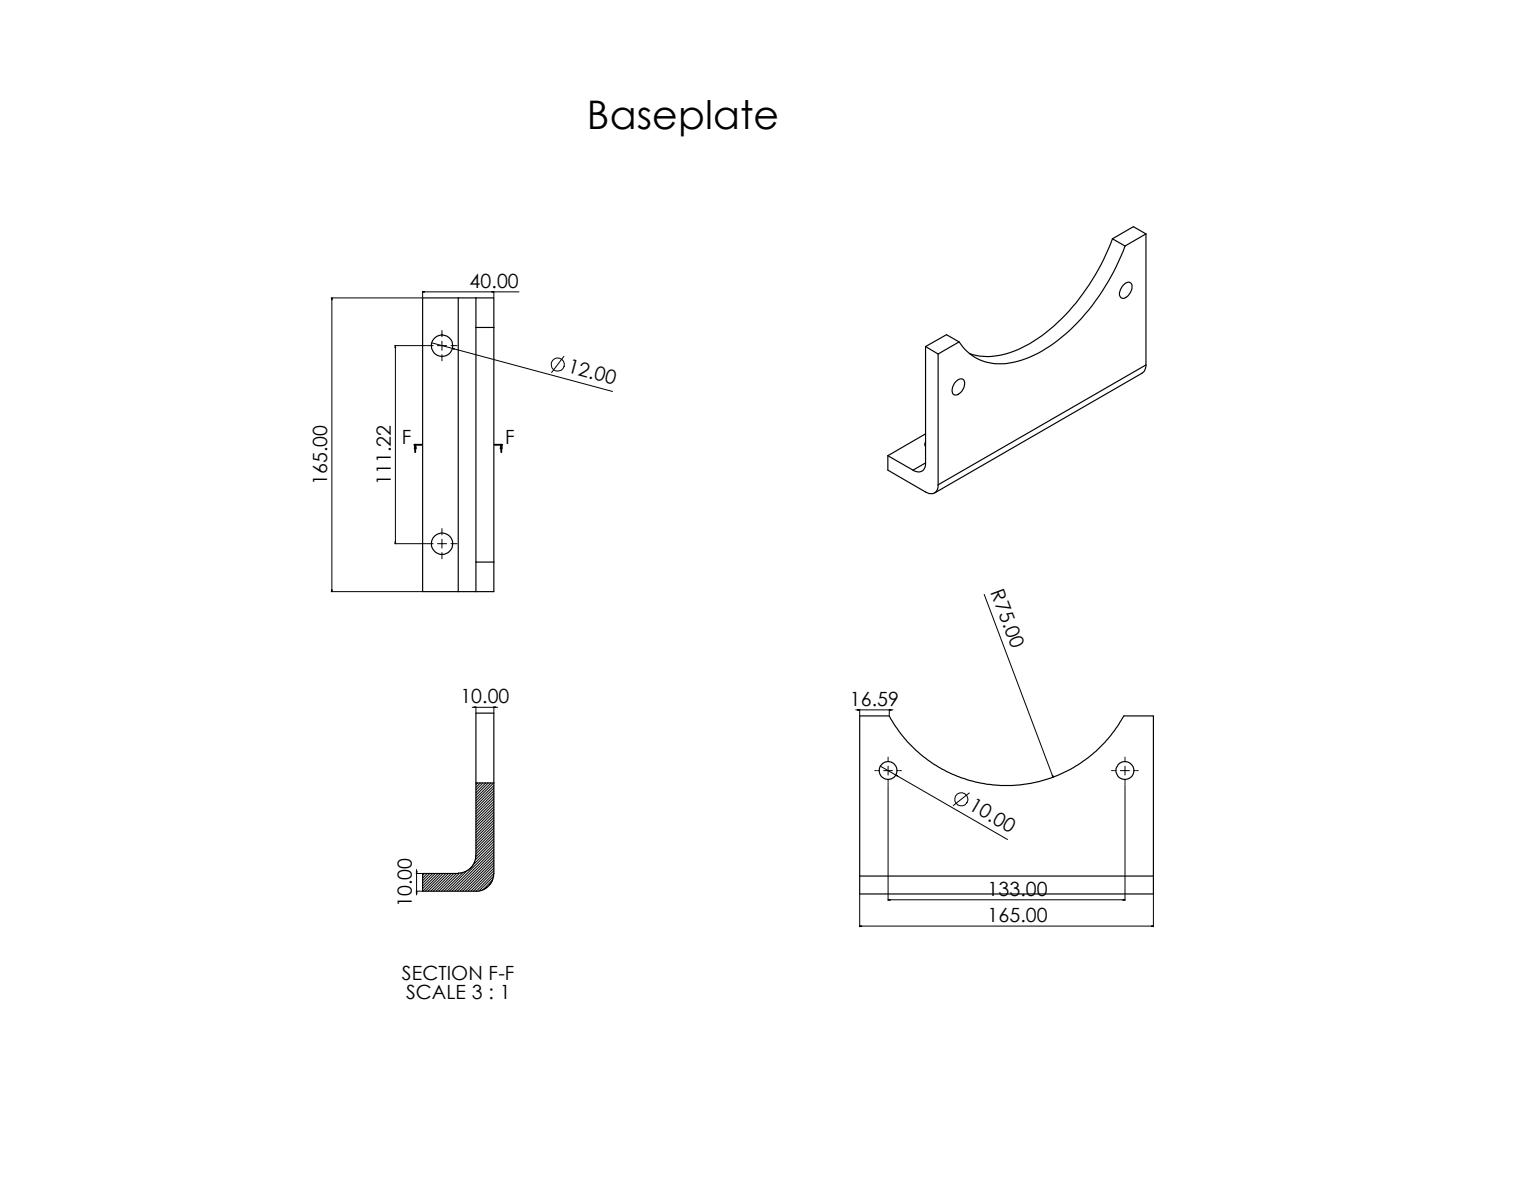
ISO-10303-21;
HEADER;
FILE_DESCRIPTION (('STEP AP214'),
    '1' );
FILE_NAME ('Baseplate.step',
    '2026-10-27T19:20:31',
    ( '' ),
    ( '' ),
    'SwSTEP 2.0',
    'SolidWorks 2025',
    '' );
FILE_SCHEMA (( 'AUTOMOTIVE_DESIGN' ));
ENDSEC;

DATA;
#22=DIRECTION ( 'NONE',  ( 0.000000000000000000, 0.000000000000000000, 1.000000000000000000 ) ) ;
#38=DIRECTION ( 'NONE',  ( -1.836970198721030427E-16, 1.000000000000000000, -1.682156097916904327E-16 ) ) ;
#169=DIRECTION ( 'NONE',  ( 0.000000000000000000, -1.000000000000000000, 0.000000000000000000 ) ) ;
#190=EDGE_CURVE ( 'NONE', #22454, #4199, #20086, .T. ) ;
#222=( GEOMETRIC_REPRESENTATION_CONTEXT ( 3 ) GLOBAL_UNCERTAINTY_ASSIGNED_CONTEXT ( ( #25788 ) ) GLOBAL_UNIT_ASSIGNED_CONTEXT ( ( #19170, #953, #19420 ) ) REPRESENTATION_CONTEXT ( 'NONE', 'WORKASPACE' ) );
#232=CIRCLE ( 'NONE', #10863, 5.000000000000004441 ) ;
#247=AXIS2_PLACEMENT_3D ( 'NONE', #22404, #17983, #169 ) ;
#303=CARTESIAN_POINT ( 'NONE',  ( 190.0000000000000000, 2.476104986517924766E-14, 4.683861624749757595E-30 ) ) ;
#341=CARTESIAN_POINT ( 'NONE',  ( 180.0000000000000000, -61.50000000000001421, 66.50000000000005684 ) ) ;
#389=EDGE_CURVE ( 'NONE', #22079, #14258, #2389, .T. ) ;
#393=VECTOR ( 'NONE', #2972, 1000.000000000000000 ) ;
#453=CARTESIAN_POINT ( 'NONE',  ( 150.0000000000000284, -135.7889608577475258, -82.49999999999998579 ) ) ;
#459=LINE ( 'NONE', #6827, #7636 ) ;
#575=PLANE ( 'NONE',  #7887 ) ;
#693=EDGE_LOOP ( 'NONE', ( #13184, #9222, #23705, #13464 ) ) ;
#761=ORIENTED_EDGE ( 'NONE', *, *, #11193, .T. ) ;
#786=ORIENTED_EDGE ( 'NONE', *, *, #16697, .F. ) ;
#795=EDGE_CURVE ( 'NONE', #24980, #854, #10474, .T. ) ;
#848=LINE ( 'NONE', #8957, #8452 ) ;
#854=VERTEX_POINT ( 'NONE', #22798 ) ;
#878=CARTESIAN_POINT ( 'NONE',  ( 160.9163046357249129, -135.7889608577475542, -55.61140153332245006 ) ) ;
#890=ORIENTED_EDGE ( 'NONE', *, *, #2098, .F. ) ;
#953=( NAMED_UNIT ( * ) PLANE_ANGLE_UNIT ( ) SI_UNIT ( $, .RADIAN. ) );
#983=DIRECTION ( 'NONE',  ( 1.000000000000000000, 1.836970198721030427E-16, -0.000000000000000000 ) ) ;
#1049=ORIENTED_EDGE ( 'NONE', *, *, #22501, .T. ) ;
#1059=LINE ( 'NONE', #1190, #21088 ) ;
#1076=DIRECTION ( 'NONE',  ( -1.303213150798907793E-16, 1.000000000000000000, -1.682156097916904081E-16 ) ) ;
#1086=VECTOR ( 'NONE', #8418, 1000.000000000000000 ) ;
#1119=ORIENTED_EDGE ( 'NONE', *, *, #1862, .F. ) ;
#1146=LINE ( 'NONE', #13362, #1967 ) ;
#1164=CARTESIAN_POINT ( 'NONE',  ( 160.9163046357249129, -135.7889608577475542, -61.61140153332246427 ) ) ;
#1190=CARTESIAN_POINT ( 'NONE',  ( 160.9163046357249129, -205.7889608577475542, 61.61140153332252112 ) ) ;
#1237=ORIENTED_EDGE ( 'NONE', *, *, #12981, .F. ) ;
#1245=EDGE_LOOP ( 'NONE', ( #24383, #1697, #17206, #26322 ) ) ;
#1290=DIRECTION ( 'NONE',  ( -1.000000000000000000, -1.836970198721030427E-16, 0.000000000000000000 ) ) ;
#1371=CYLINDRICAL_SURFACE ( 'NONE', #14023, 5.000000000000004441 ) ;
#1437=AXIS2_PLACEMENT_3D ( 'NONE', #19135, #5044, #3043 ) ;
#1446=LINE ( 'NONE', #23782, #16395 ) ;
#1451=FACE_OUTER_BOUND ( 'NONE', #20749, .T. ) ;
#1462=DIRECTION ( 'NONE',  ( 1.000000000000000000, 1.836970198721030427E-16, -0.000000000000000000 ) ) ;
#1499=EDGE_CURVE ( 'NONE', #1963, #23636, #7438, .T. ) ;
#1524=CIRCLE ( 'NONE', #247, 9.999999999999994671 ) ;
#1616=DIRECTION ( 'NONE',  ( -5.098616525425841937E-32, 2.775557561562890858E-16, 1.000000000000000000 ) ) ;
#1627=FACE_OUTER_BOUND ( 'NONE', #2486, .T. ) ;
#1641=AXIS2_PLACEMENT_3D ( 'NONE', #21190, #23317, #16661 ) ;
#1644=CARTESIAN_POINT ( 'NONE',  ( 180.0000000000000284, -125.7889608577475116, 82.50000000000001421 ) ) ;
#1661=ORIENTED_EDGE ( 'NONE', *, *, #9798, .F. ) ;
#1697=ORIENTED_EDGE ( 'NONE', *, *, #15786, .F. ) ;
#1720=SHAPE_DEFINITION_REPRESENTATION ( #22072, #14572 ) ;
#1730=CARTESIAN_POINT ( 'NONE',  ( 150.0000000000000284, -125.7889608577475116, 82.50000000000001421 ) ) ;
#1737=CIRCLE ( 'NONE', #16606, 6.000000000000005329 ) ;
#1764=ADVANCED_FACE ( 'NONE', ( #15599, #23724, #21735 ), #7614, .F. ) ;
#1799=CIRCLE ( 'NONE', #3481, 6.000000000000019540 ) ;
#1819=ADVANCED_FACE ( 'NONE', ( #21360 ), #3129, .F. ) ;
#1862=EDGE_CURVE ( 'NONE', #16337, #25804, #232, .T. ) ;
#1901=ORIENTED_EDGE ( 'NONE', *, *, #389, .F. ) ;
#1963=VERTEX_POINT ( 'NONE', #1164 ) ;
#1967=VECTOR ( 'NONE', #9633, 1000.000000000000000 ) ;
#1981=VECTOR ( 'NONE', #5648, 1000.000000000000000 ) ;
#1984=VERTEX_POINT ( 'NONE', #7261 ) ;
#1994=DIRECTION ( 'NONE',  ( 2.985653255390529422E-32, -4.182618615277681568E-16, 1.000000000000000000 ) ) ;
#2001=EDGE_CURVE ( 'NONE', #23636, #1963, #4068, .T. ) ;
#2032=CARTESIAN_POINT ( 'NONE',  ( 160.9163046357249129, -125.7889608577475684, -55.61140153332245006 ) ) ;
#2071=CARTESIAN_POINT ( 'NONE',  ( 180.0000000000000284, -115.7889608577475258, 82.50000000000000000 ) ) ;
#2098=EDGE_CURVE ( 'NONE', #3856, #1984, #3667, .T. ) ;
#2174=DIRECTION ( 'NONE',  ( 0.000000000000000000, 0.000000000000000000, 1.000000000000000000 ) ) ;
#2186=VECTOR ( 'NONE', #25982, 1000.000000000000000 ) ;
#2193=CIRCLE ( 'NONE', #17641, 10.00000000000000888 ) ;
#2273=PLANE ( 'NONE',  #23836 ) ;
#2302=DIRECTION ( 'NONE',  ( 1.000000000000000000, 1.836970198721030427E-16, -0.000000000000000000 ) ) ;
#2313=EDGE_CURVE ( 'NONE', #25993, #2419, #22542, .T. ) ;
#2389=CIRCLE ( 'NONE', #20666, 6.000000000000019540 ) ;
#2419=VERTEX_POINT ( 'NONE', #14277 ) ;
#2425=VERTEX_POINT ( 'NONE', #453 ) ;
#2486=EDGE_LOOP ( 'NONE', ( #15483, #4393, #761, #12919 ) ) ;
#2514=CARTESIAN_POINT ( 'NONE',  ( 190.0000000000000000, -66.50000000000001421, -66.50000000000005684 ) ) ;
#2541=DIRECTION ( 'NONE',  ( 0.000000000000000000, -1.000000000000000000, 0.000000000000000000 ) ) ;
#2542=CARTESIAN_POINT ( 'NONE',  ( 190.0000000000000284, -125.7889608577475400, 2.115966675574909200E-14 ) ) ;
#2598=ADVANCED_FACE ( 'NONE', ( #23153 ), #20895, .F. ) ;
#2627=AXIS2_PLACEMENT_3D ( 'NONE', #12406, #2302, #18529 ) ;
#2757=EDGE_LOOP ( 'NONE', ( #3114, #1049, #11674, #13097 ) ) ;
#2799=AXIS2_PLACEMENT_3D ( 'NONE', #21130, #9017, #25385 ) ;
#2813=PRODUCT_DEFINITION_FORMATION_WITH_SPECIFIED_SOURCE ( 'ANY', '', #15879, .NOT_KNOWN. ) ;
#2815=CARTESIAN_POINT ( 'NONE',  ( 180.0000000000000000, 2.292407966645821729E-14, 4.683861624749757595E-30 ) ) ;
#2925=CARTESIAN_POINT ( 'NONE',  ( 180.0000000000000284, -125.7889608577475684, -82.49999999999998579 ) ) ;
#2972=DIRECTION ( 'NONE',  ( -1.303213150798907793E-16, 1.000000000000000000, -1.682156097916904081E-16 ) ) ;
#2985=EDGE_CURVE ( 'NONE', #23734, #20976, #1059, .T. ) ;
#3043=DIRECTION ( 'NONE',  ( 0.000000000000000000, 0.000000000000000000, 1.000000000000000000 ) ) ;
#3114=ORIENTED_EDGE ( 'NONE', *, *, #15003, .T. ) ;
#3129=CYLINDRICAL_SURFACE ( 'NONE', #16804, 6.000000000000019540 ) ;
#3149=ADVANCED_FACE ( 'NONE', ( #9918 ), #11915, .F. ) ;
#3162=FACE_BOUND ( 'NONE', #7335, .T. ) ;
#3231=CARTESIAN_POINT ( 'NONE',  ( 180.0000000000000000, -66.50000000000001421, 66.50000000000005684 ) ) ;
#3239=VERTEX_POINT ( 'NONE', #4611 ) ;
#3268=AXIS2_PLACEMENT_3D ( 'NONE', #24504, #16507, #2541 ) ;
#3286=PLANE ( 'NONE',  #16622 ) ;
#3391=EDGE_CURVE ( 'NONE', #22320, #25804, #8962, .T. ) ;
#3481=AXIS2_PLACEMENT_3D ( 'NONE', #7276, #3549, #15638 ) ;
#3488=DIRECTION ( 'NONE',  ( 0.000000000000000000, 1.000000000000000000, 0.000000000000000000 ) ) ;
#3495=ORIENTED_EDGE ( 'NONE', *, *, #4923, .T. ) ;
#3511=CARTESIAN_POINT ( 'NONE',  ( 150.0000000000000284, -125.7889608577475116, 82.50000000000001421 ) ) ;
#3549=DIRECTION ( 'NONE',  ( -1.303213150798907793E-16, 1.000000000000000000, -1.682156097916904081E-16 ) ) ;
#3564=LINE ( 'NONE', #25933, #6385 ) ;
#3614=DIRECTION ( 'NONE',  ( -1.303213150798907793E-16, 1.000000000000000000, -1.682156097916904081E-16 ) ) ;
#3644=AXIS2_PLACEMENT_3D ( 'NONE', #26029, #19888, #19624 ) ;
#3654=AXIS2_PLACEMENT_3D ( 'NONE', #4347, #5933, #18024 ) ;
#3661=CARTESIAN_POINT ( 'NONE',  ( 180.0000000000000000, -35.78896085774750446, -65.91016826501511616 ) ) ;
#3667=LINE ( 'NONE', #5931, #9143 ) ;
#3723=VERTEX_POINT ( 'NONE', #7849 ) ;
#3849=CIRCLE ( 'NONE', #7183, 5.000000000000004441 ) ;
#3856=VERTEX_POINT ( 'NONE', #7413 ) ;
#3876=EDGE_CURVE ( 'NONE', #9443, #22454, #1446, .T. ) ;
#3925=CARTESIAN_POINT ( 'NONE',  ( 150.0000000000000284, -125.7889608577475116, 82.50000000000001421 ) ) ;
#3957=EDGE_LOOP ( 'NONE', ( #25081, #3495, #786, #25524, #5205, #9062, #4826, #21169 ) ) ;
#3989=ORIENTED_EDGE ( 'NONE', *, *, #9879, .F. ) ;
#4021=ORIENTED_EDGE ( 'NONE', *, *, #11906, .T. ) ;
#4064=( GEOMETRIC_REPRESENTATION_CONTEXT ( 3 ) GLOBAL_UNCERTAINTY_ASSIGNED_CONTEXT ( ( #15216 ) ) GLOBAL_UNIT_ASSIGNED_CONTEXT ( ( #10800, #10528, #18506 ) ) REPRESENTATION_CONTEXT ( 'NONE', 'WORKASPACE' ) );
#4068=CIRCLE ( 'NONE', #2799, 6.000000000000005329 ) ;
#4134=ORIENTED_EDGE ( 'NONE', *, *, #15447, .T. ) ;
#4137=DIRECTION ( 'NONE',  ( 0.000000000000000000, -1.682156097916903834E-16, -1.000000000000000000 ) ) ;
#4168=VERTEX_POINT ( 'NONE', #3925 ) ;
#4199=VERTEX_POINT ( 'NONE', #16543 ) ;
#4234=DIRECTION ( 'NONE',  ( -1.303213150798907793E-16, 1.000000000000000000, -1.682156097916904081E-16 ) ) ;
#4284=FACE_OUTER_BOUND ( 'NONE', #10394, .T. ) ;
#4347=CARTESIAN_POINT ( 'NONE',  ( 169.9999999999999716, -115.7889608577475258, 82.50000000000001421 ) ) ;
#4393=ORIENTED_EDGE ( 'NONE', *, *, #23125, .F. ) ;
#4439=CYLINDRICAL_SURFACE ( 'NONE', #5169, 74.99999999999995737 ) ;
#4459=EDGE_LOOP ( 'NONE', ( #13810, #22818, #22074, #18648 ) ) ;
#4495=DIRECTION ( 'NONE',  ( 1.000000000000000000, 1.303213150798907793E-16, 2.465190328815661892E-32 ) ) ;
#4549=LINE ( 'NONE', #14377, #15153 ) ;
#4571=CARTESIAN_POINT ( 'NONE',  ( 190.0000000000000000, 4.765939974807309500E-14, 82.49999999999997158 ) ) ;
#4580=DIRECTION ( 'NONE',  ( 1.000000000000000000, 1.303213150798907793E-16, 2.465190328815661892E-32 ) ) ;
#4604=ADVANCED_FACE ( 'NONE', ( #15815 ), #15950, .F. ) ;
#4611=CARTESIAN_POINT ( 'NONE',  ( 180.0000000000000284, -135.7889608577475542, -82.49999999999998579 ) ) ;
#4631=DIRECTION ( 'NONE',  ( 2.985653255390529422E-32, -4.182618615277681568E-16, 1.000000000000000000 ) ) ;
#4666=DIRECTION ( 'NONE',  ( 1.000000000000000000, 0.000000000000000000, -0.000000000000000000 ) ) ;
#4725=CARTESIAN_POINT ( 'NONE',  ( 160.9163046357249129, -125.7889608577475400, 55.61140153332248559 ) ) ;
#4826=ORIENTED_EDGE ( 'NONE', *, *, #15003, .F. ) ;
#4923=EDGE_CURVE ( 'NONE', #1984, #6082, #2193, .T. ) ;
#4973=EDGE_CURVE ( 'NONE', #9342, #8967, #1524, .T. ) ;
#5044=DIRECTION ( 'NONE',  ( -1.303213150798907793E-16, 1.000000000000000000, -1.682156097916904081E-16 ) ) ;
#5079=EDGE_LOOP ( 'NONE', ( #1119, #10639 ) ) ;
#5169=AXIS2_PLACEMENT_3D ( 'NONE', #10548, #21194, #9079 ) ;
#5180=AXIS2_PLACEMENT_3D ( 'NONE', #15679, #23804, #23309 ) ;
#5205=ORIENTED_EDGE ( 'NONE', *, *, #15010, .T. ) ;
#5263=ORIENTED_EDGE ( 'NONE', *, *, #25351, .T. ) ;
#5362=VERTEX_POINT ( 'NONE', #20369 ) ;
#5374=CARTESIAN_POINT ( 'NONE',  ( 160.9163046357249129, -125.7889608577475684, -61.61140153332246427 ) ) ;
#5379=DIRECTION ( 'NONE',  ( -1.000000000000000000, 0.000000000000000000, 0.000000000000000000 ) ) ;
#5505=DIRECTION ( 'NONE',  ( -1.836970198721030427E-16, 1.000000000000000000, -1.682156097916904327E-16 ) ) ;
#5624=DIRECTION ( 'NONE',  ( 1.000000000000000000, 1.303213150798907793E-16, 2.465190328815661892E-32 ) ) ;
#5648=DIRECTION ( 'NONE',  ( 1.303213150798907793E-16, -1.000000000000000000, 0.000000000000000000 ) ) ;
#5684=FACE_OUTER_BOUND ( 'NONE', #14455, .T. ) ;
#5699=PRODUCT_CONTEXT ( 'NONE', #16389, 'mechanical' ) ;
#5749=EDGE_CURVE ( 'NONE', #9443, #10429, #17877, .T. ) ;
#5767=DIRECTION ( 'NONE',  ( 0.000000000000000000, 0.000000000000000000, 1.000000000000000000 ) ) ;
#5770=VECTOR ( 'NONE', #24556, 1000.000000000000000 ) ;
#5864=DIRECTION ( 'NONE',  ( 0.000000000000000000, -4.182618615277681568E-16, 1.000000000000000000 ) ) ;
#5875=LINE ( 'NONE', #15974, #2186 ) ;
#5931=CARTESIAN_POINT ( 'NONE',  ( 180.0000000000000284, -135.7889608577475258, 82.50000000000001421 ) ) ;
#5933=DIRECTION ( 'NONE',  ( 4.657398277317546459E-32, -1.682156097916904081E-16, -1.000000000000000000 ) ) ;
#5949=CIRCLE ( 'NONE', #22097, 74.99999999999995737 ) ;
#5966=DIRECTION ( 'NONE',  ( -4.657398277317547006E-32, 1.682156097916904327E-16, 1.000000000000000000 ) ) ;
#5971=EDGE_CURVE ( 'NONE', #2425, #3856, #1146, .T. ) ;
#6082=VERTEX_POINT ( 'NONE', #13338 ) ;
#6100=DIRECTION ( 'NONE',  ( 0.000000000000000000, -4.182618615277681568E-16, -1.000000000000000000 ) ) ;
#6106=ORIENTED_EDGE ( 'NONE', *, *, #24953, .T. ) ;
#6111=CARTESIAN_POINT ( 'NONE',  ( 190.0000000000000000, -35.78896085774753288, -1.496915739050591872E-14 ) ) ;
#6142=DIRECTION ( 'NONE',  ( 0.000000000000000000, 0.000000000000000000, -1.000000000000000000 ) ) ;
#6240=EDGE_LOOP ( 'NONE', ( #1237, #23465, #23167, #18848 ) ) ;
#6283=CARTESIAN_POINT ( 'NONE',  ( 169.9999999999999716, -115.7889608577475542, -82.49999999999998579 ) ) ;
#6370=EDGE_CURVE ( 'NONE', #21146, #2419, #9439, .T. ) ;
#6385=VECTOR ( 'NONE', #24052, 1000.000000000000000 ) ;
#6386=DIRECTION ( 'NONE',  ( -1.836970198721030427E-16, 1.000000000000000000, 4.182618615277681568E-16 ) ) ;
#6460=VECTOR ( 'NONE', #12832, 1000.000000000000000 ) ;
#6476=CARTESIAN_POINT ( 'NONE',  ( 180.0000000000000000, -35.78896085774753288, -1.496915739050591872E-14 ) ) ;
#6530=ORIENTED_EDGE ( 'NONE', *, *, #15786, .T. ) ;
#6537=ORIENTED_EDGE ( 'NONE', *, *, #16385, .F. ) ;
#6548=DIRECTION ( 'NONE',  ( 0.000000000000000000, -1.000000000000000000, 0.000000000000000000 ) ) ;
#6553=CARTESIAN_POINT ( 'NONE',  ( 160.9163046357249129, -205.7889608577475542, -61.61140153332245006 ) ) ;
#6633=EDGE_CURVE ( 'NONE', #25845, #3723, #11178, .T. ) ;
#6677=DIRECTION ( 'NONE',  ( 1.303213150798907793E-16, -1.000000000000000000, 0.000000000000000000 ) ) ;
#6764=ORIENTED_EDGE ( 'NONE', *, *, #9798, .T. ) ;
#6805=DIRECTION ( 'NONE',  ( 7.916033913021854848E-32, -4.182618615277681568E-16, -1.000000000000000000 ) ) ;
#6827=CARTESIAN_POINT ( 'NONE',  ( 180.0000000000000000, -35.78896085774750446, -65.91016826501511616 ) ) ;
#6831=DIRECTION ( 'NONE',  ( 0.000000000000000000, 0.000000000000000000, 1.000000000000000000 ) ) ;
#6832=ORIENTED_EDGE ( 'NONE', *, *, #19629, .F. ) ;
#6873=DIRECTION ( 'NONE',  ( 0.000000000000000000, -1.000000000000000000, 0.000000000000000000 ) ) ;
#6895=ORIENTED_EDGE ( 'NONE', *, *, #25351, .F. ) ;
#6961=EDGE_CURVE ( 'NONE', #23006, #20872, #25251, .T. ) ;
#7117=ADVANCED_FACE ( 'NONE', ( #21143 ), #11025, .F. ) ;
#7183=AXIS2_PLACEMENT_3D ( 'NONE', #15307, #11315, #19555 ) ;
#7212=ORIENTED_EDGE ( 'NONE', *, *, #2001, .T. ) ;
#7261=CARTESIAN_POINT ( 'NONE',  ( 180.0000000000000284, -135.7889608577475258, 82.50000000000001421 ) ) ;
#7276=CARTESIAN_POINT ( 'NONE',  ( 160.9163046357249129, -125.7889608577475684, -55.61140153332245006 ) ) ;
#7335=EDGE_LOOP ( 'NONE', ( #7212, #11305 ) ) ;
#7413=CARTESIAN_POINT ( 'NONE',  ( 150.0000000000000284, -135.7889608577475258, 82.50000000000001421 ) ) ;
#7435=ORIENTED_EDGE ( 'NONE', *, *, #19387, .F. ) ;
#7438=CIRCLE ( 'NONE', #15506, 6.000000000000005329 ) ;
#7494=CARTESIAN_POINT ( 'NONE',  ( 150.0000000000000284, -135.7889608577475258, -82.49999999999998579 ) ) ;
#7581=VECTOR ( 'NONE', #14565, 1000.000000000000000 ) ;
#7600=EDGE_LOOP ( 'NONE', ( #11859, #16068 ) ) ;
#7614=PLANE ( 'NONE',  #22333 ) ;
#7636=VECTOR ( 'NONE', #16678, 1000.000000000000000 ) ;
#7697=VECTOR ( 'NONE', #4137, 1000.000000000000000 ) ;
#7720=ORIENTED_EDGE ( 'NONE', *, *, #2001, .F. ) ;
#7748=FACE_OUTER_BOUND ( 'NONE', #16341, .T. ) ;
#7759=EDGE_CURVE ( 'NONE', #20976, #3723, #21716, .T. ) ;
#7849=CARTESIAN_POINT ( 'NONE',  ( 160.9163046357249129, -125.7889608577475400, 49.61140153332247138 ) ) ;
#7854=DIRECTION ( 'NONE',  ( -0.000000000000000000, 0.000000000000000000, 1.000000000000000000 ) ) ;
#7887=AXIS2_PLACEMENT_3D ( 'NONE', #303, #10950, #6677 ) ;
#7891=VECTOR ( 'NONE', #1462, 1000.000000000000000 ) ;
#7955=ORIENTED_EDGE ( 'NONE', *, *, #21219, .T. ) ;
#7994=CARTESIAN_POINT ( 'NONE',  ( 0.000000000000000000, 0.000000000000000000, 0.000000000000000000 ) ) ;
#8014=DIRECTION ( 'NONE',  ( -1.000000000000000000, 0.000000000000000000, 0.000000000000000000 ) ) ;
#8108=AXIS2_PLACEMENT_3D ( 'NONE', #10204, #4234, #16713 ) ;
#8143=CARTESIAN_POINT ( 'NONE',  ( 160.9163046357249129, -125.7889608577475400, 61.61140153332250691 ) ) ;
#8304=CARTESIAN_POINT ( 'NONE',  ( 180.0000000000000284, -135.7889608577475542, -82.49999999999998579 ) ) ;
#8312=LINE ( 'NONE', #341, #7581 ) ;
#8385=DIRECTION ( 'NONE',  ( 1.000000000000000000, 1.303213150798907793E-16, 2.465190328815661892E-32 ) ) ;
#8418=DIRECTION ( 'NONE',  ( 7.916033913021854848E-32, -4.182618615277681568E-16, -1.000000000000000000 ) ) ;
#8452=VECTOR ( 'NONE', #4580, 1000.000000000000000 ) ;
#8602=ORIENTED_EDGE ( 'NONE', *, *, #19395, .T. ) ;
#8716=DIRECTION ( 'NONE',  ( 1.000000000000000000, 1.836970198721030427E-16, -0.000000000000000000 ) ) ;
#8731=AXIS2_PLACEMENT_3D ( 'NONE', #16754, #23028, #4666 ) ;
#8759=ORIENTED_EDGE ( 'NONE', *, *, #18586, .T. ) ;
#8808=CARTESIAN_POINT ( 'NONE',  ( 180.0000000000000000, -35.78896085774753288, 1.496915739050593134E-14 ) ) ;
#8875=CARTESIAN_POINT ( 'NONE',  ( 180.0000000000000000, -66.50000000000001421, -66.50000000000005684 ) ) ;
#8940=ORIENTED_EDGE ( 'NONE', *, *, #19486, .T. ) ;
#8957=CARTESIAN_POINT ( 'NONE',  ( 150.0000000000000284, -125.7889608577475400, -82.49999999999998579 ) ) ;
#8962=LINE ( 'NONE', #19201, #20220 ) ;
#8967=VERTEX_POINT ( 'NONE', #24525 ) ;
#9017=DIRECTION ( 'NONE',  ( -1.836970198721030427E-16, 1.000000000000000000, -1.682156097916904327E-16 ) ) ;
#9062=ORIENTED_EDGE ( 'NONE', *, *, #4973, .T. ) ;
#9079=DIRECTION ( 'NONE',  ( 0.000000000000000000, 1.000000000000000000, 0.000000000000000000 ) ) ;
#9091=LINE ( 'NONE', #19579, #11139 ) ;
#9093=EDGE_LOOP ( 'NONE', ( #12262, #7720, #4021, #18474 ) ) ;
#9097=ORIENTED_EDGE ( 'NONE', *, *, #6370, .F. ) ;
#9143=VECTOR ( 'NONE', #26035, 1000.000000000000000 ) ;
#9200=CARTESIAN_POINT ( 'NONE',  ( 180.0000000000000284, -115.7889608577475542, -82.49999999999998579 ) ) ;
#9218=LINE ( 'NONE', #19451, #22619 ) ;
#9222=ORIENTED_EDGE ( 'NONE', *, *, #3391, .T. ) ;
#9335=DIRECTION ( 'NONE',  ( 0.000000000000000000, -1.000000000000000000, 2.775557561562890858E-16 ) ) ;
#9342=VERTEX_POINT ( 'NONE', #2071 ) ;
#9439=LINE ( 'NONE', #15299, #7891 ) ;
#9443=VERTEX_POINT ( 'NONE', #20425 ) ;
#9450=CARTESIAN_POINT ( 'NONE',  ( 160.9163046357249129, -205.7889608577475542, -55.61140153332243585 ) ) ;
#9468=DIRECTION ( 'NONE',  ( 1.000000000000000000, 1.303213150798907793E-16, 2.465190328815661892E-32 ) ) ;
#9471=ORIENTED_EDGE ( 'NONE', *, *, #10438, .T. ) ;
#9546=DIRECTION ( 'NONE',  ( 1.000000000000000000, 1.836970198721030427E-16, -0.000000000000000000 ) ) ;
#9626=DIRECTION ( 'NONE',  ( 1.303213150798907793E-16, -1.000000000000000000, 1.682156097916904081E-16 ) ) ;
#9633=DIRECTION ( 'NONE',  ( -0.000000000000000000, -0.000000000000000000, 1.000000000000000000 ) ) ;
#9664=ORIENTED_EDGE ( 'NONE', *, *, #19395, .F. ) ;
#9686=CARTESIAN_POINT ( 'NONE',  ( 160.9163046357249129, -135.7889608577475542, -49.61140153332242875 ) ) ;
#9798=EDGE_CURVE ( 'NONE', #2419, #4199, #5949, .T. ) ;
#9866=PLANE ( 'NONE',  #23792 ) ;
#9874=ORIENTED_EDGE ( 'NONE', *, *, #12981, .T. ) ;
#9879=EDGE_CURVE ( 'NONE', #21371, #10429, #18203, .T. ) ;
#9918=FACE_OUTER_BOUND ( 'NONE', #13584, .T. ) ;
#10018=DIRECTION ( 'NONE',  ( 1.000000000000000000, 1.836970198721030427E-16, -0.000000000000000000 ) ) ;
#10042=EDGE_CURVE ( 'NONE', #25804, #16337, #15286, .T. ) ;
#10101=EDGE_CURVE ( 'NONE', #3856, #4168, #24793, .T. ) ;
#10204=CARTESIAN_POINT ( 'NONE',  ( 160.9163046357249129, -125.7889608577475400, 55.61140153332248559 ) ) ;
#10283=DIRECTION ( 'NONE',  ( -5.098616525425841937E-32, 2.775557561562890858E-16, 1.000000000000000000 ) ) ;
#10394=EDGE_LOOP ( 'NONE', ( #13153, #19009, #23266, #5263 ) ) ;
#10399=EDGE_LOOP ( 'NONE', ( #17360, #16816, #26219, #13058 ) ) ;
#10429=VERTEX_POINT ( 'NONE', #9200 ) ;
#10438=EDGE_CURVE ( 'NONE', #21905, #25993, #25964, .T. ) ;
#10459=VECTOR ( 'NONE', #1994, 1000.000000000000000 ) ;
#10474=CIRCLE ( 'NONE', #13836, 5.000000000000004441 ) ;
#10528=( NAMED_UNIT ( * ) PLANE_ANGLE_UNIT ( ) SI_UNIT ( $, .RADIAN. ) );
#10548=CARTESIAN_POINT ( 'NONE',  ( 180.0000000000000000, 6.980486755139914804E-14, 0.000000000000000000 ) ) ;
#10573=LINE ( 'NONE', #8304, #5770 ) ;
#10629=DIRECTION ( 'NONE',  ( 1.000000000000000000, 1.303213150798907793E-16, 2.465190328815661892E-32 ) ) ;
#10639=ORIENTED_EDGE ( 'NONE', *, *, #10042, .F. ) ;
#10659=CARTESIAN_POINT ( 'NONE',  ( 180.0000000000000000, 4.582242954935206147E-14, 82.49999999999997158 ) ) ;
#10668=VERTEX_POINT ( 'NONE', #23907 ) ;
#10673=ORIENTED_EDGE ( 'NONE', *, *, #16393, .T. ) ;
#10687=DIRECTION ( 'NONE',  ( 1.000000000000000000, 1.303213150798907793E-16, 2.465190328815661892E-32 ) ) ;
#10800=( LENGTH_UNIT ( ) NAMED_UNIT ( * ) SI_UNIT ( .MILLI., .METRE. ) );
#10860=EDGE_LOOP ( 'NONE', ( #7435, #25551, #20916, #11593 ) ) ;
#10863=AXIS2_PLACEMENT_3D ( 'NONE', #11258, #11013, #13506 ) ;
#10950=DIRECTION ( 'NONE',  ( -1.000000000000000000, -1.303213150798907793E-16, -2.465190328815661892E-32 ) ) ;
#10969=EDGE_LOOP ( 'NONE', ( #6764, #6895, #23580, #12691 ) ) ;
#11013=DIRECTION ( 'NONE',  ( 1.000000000000000000, 1.303213150798907793E-16, 2.465190328815661892E-32 ) ) ;
#11025=CYLINDRICAL_SURFACE ( 'NONE', #1437, 6.000000000000019540 ) ;
#11069=CARTESIAN_POINT ( 'NONE',  ( 190.0000000000000000, -71.50000000000002842, -66.50000000000005684 ) ) ;
#11139=VECTOR ( 'NONE', #25591, 1000.000000000000000 ) ;
#11178=LINE ( 'NONE', #19293, #11496 ) ;
#11193=EDGE_CURVE ( 'NONE', #10668, #16337, #8312, .T. ) ;
#11194=DIRECTION ( 'NONE',  ( 1.000000000000000000, 1.836970198721030427E-16, -0.000000000000000000 ) ) ;
#11214=APPLICATION_CONTEXT ( 'automotive_design' ) ;
#11258=CARTESIAN_POINT ( 'NONE',  ( 190.0000000000000000, -66.50000000000001421, 66.50000000000005684 ) ) ;
#11305=ORIENTED_EDGE ( 'NONE', *, *, #1499, .T. ) ;
#11315=DIRECTION ( 'NONE',  ( 1.000000000000000000, 1.303213150798907793E-16, 2.465190328815661892E-32 ) ) ;
#11333=ORIENTED_EDGE ( 'NONE', *, *, #24254, .F. ) ;
#11346=ADVANCED_FACE ( 'NONE', ( #20832 ), #23100, .F. ) ;
#11348=CARTESIAN_POINT ( 'NONE',  ( 190.0000000000000000, 7.164183775012017527E-14, 0.000000000000000000 ) ) ;
#11455=DIRECTION ( 'NONE',  ( 1.000000000000000000, 1.836970198721030427E-16, -0.000000000000000000 ) ) ;
#11496=VECTOR ( 'NONE', #1076, 1000.000000000000000 ) ;
#11556=ORIENTED_EDGE ( 'NONE', *, *, #6961, .T. ) ;
#11592=PRODUCT_DEFINITION ( 'UNKNOWN', '', #2813, #25476 ) ;
#11593=ORIENTED_EDGE ( 'NONE', *, *, #21349, .T. ) ;
#11622=AXIS2_PLACEMENT_3D ( 'NONE', #2514, #10629, #18741 ) ;
#11674=ORIENTED_EDGE ( 'NONE', *, *, #11905, .F. ) ;
#11859=ORIENTED_EDGE ( 'NONE', *, *, #7759, .F. ) ;
#11888=VECTOR ( 'NONE', #15189, 1000.000000000000000 ) ;
#11905=EDGE_CURVE ( 'NONE', #5362, #21371, #848, .T. ) ;
#11906=EDGE_CURVE ( 'NONE', #23636, #22079, #21327, .T. ) ;
#11915=CYLINDRICAL_SURFACE ( 'NONE', #3654, 9.999999999999994671 ) ;
#11923=ORIENTED_EDGE ( 'NONE', *, *, #190, .T. ) ;
#11985=FACE_BOUND ( 'NONE', #25425, .T. ) ;
#12021=DIRECTION ( 'NONE',  ( -1.303213150798907793E-16, 1.000000000000000000, -1.682156097916904081E-16 ) ) ;
#12062=EDGE_CURVE ( 'NONE', #1963, #14258, #14664, .T. ) ;
#12243=ADVANCED_FACE ( 'NONE', ( #25703 ), #21572, .T. ) ;
#12262=ORIENTED_EDGE ( 'NONE', *, *, #12062, .F. ) ;
#12294=AXIS2_PLACEMENT_3D ( 'NONE', #24193, #5966, #14077 ) ;
#12350=EDGE_LOOP ( 'NONE', ( #24342, #18102 ) ) ;
#12377=LINE ( 'NONE', #10659, #22411 ) ;
#12390=CIRCLE ( 'NONE', #5180, 5.000000000000004441 ) ;
#12406=CARTESIAN_POINT ( 'NONE',  ( 180.0000000000000000, -66.50000000000001421, -66.50000000000005684 ) ) ;
#12507=DIRECTION ( 'NONE',  ( 4.657398277317547006E-32, -1.682156097916904081E-16, -1.000000000000000000 ) ) ;
#12560=ADVANCED_FACE ( 'NONE', ( #4284 ), #2273, .T. ) ;
#12646=DIRECTION ( 'NONE',  ( 1.303213150798907793E-16, -1.000000000000000000, 0.000000000000000000 ) ) ;
#12689=CARTESIAN_POINT ( 'NONE',  ( 190.0000000000000000, 2.476104986517924766E-14, -82.49999999999998579 ) ) ;
#12691=ORIENTED_EDGE ( 'NONE', *, *, #6370, .T. ) ;
#12832=DIRECTION ( 'NONE',  ( 1.303213150798907793E-16, -1.000000000000000000, 0.000000000000000000 ) ) ;
#12919=ORIENTED_EDGE ( 'NONE', *, *, #1862, .T. ) ;
#12932=VERTEX_POINT ( 'NONE', #20531 ) ;
#12970=LINE ( 'NONE', #13103, #16827 ) ;
#12981=EDGE_CURVE ( 'NONE', #25845, #23734, #1737, .T. ) ;
#13058=ORIENTED_EDGE ( 'NONE', *, *, #16393, .F. ) ;
#13083=CARTESIAN_POINT ( 'NONE',  ( 160.9163046357249129, -205.7889608577475542, -49.61140153332241454 ) ) ;
#13097=ORIENTED_EDGE ( 'NONE', *, *, #21816, .F. ) ;
#13103=CARTESIAN_POINT ( 'NONE',  ( 180.0000000000000284, -135.7889608577475542, 2.284182285366599633E-14 ) ) ;
#13153=ORIENTED_EDGE ( 'NONE', *, *, #190, .F. ) ;
#13184=ORIENTED_EDGE ( 'NONE', *, *, #19486, .F. ) ;
#13218=ADVANCED_FACE ( 'NONE', ( #24662 ), #22535, .F. ) ;
#13220=ADVANCED_FACE ( 'NONE', ( #16534 ), #4439, .F. ) ;
#13306=ORIENTED_EDGE ( 'NONE', *, *, #3876, .T. ) ;
#13310=ORIENTED_EDGE ( 'NONE', *, *, #13921, .F. ) ;
#13338=CARTESIAN_POINT ( 'NONE',  ( 190.0000000000000284, -125.7889608577475400, 82.50000000000001421 ) ) ;
#13362=CARTESIAN_POINT ( 'NONE',  ( 150.0000000000000284, -135.7889608577475258, 82.50000000000001421 ) ) ;
#13464=ORIENTED_EDGE ( 'NONE', *, *, #11193, .F. ) ;
#13506=DIRECTION ( 'NONE',  ( 0.000000000000000000, -1.000000000000000000, 0.000000000000000000 ) ) ;
#13529=DIRECTION ( 'NONE',  ( 1.000000000000000000, 0.000000000000000000, 0.000000000000000000 ) ) ;
#13555=AXIS2_PLACEMENT_3D ( 'NONE', #22208, #26070, #6100 ) ;
#13584=EDGE_LOOP ( 'NONE', ( #24680, #9664, #3989, #15043 ) ) ;
#13687=ORIENTED_EDGE ( 'NONE', *, *, #2313, .F. ) ;
#13810=ORIENTED_EDGE ( 'NONE', *, *, #10101, .T. ) ;
#13836=AXIS2_PLACEMENT_3D ( 'NONE', #24796, #10687, #6548 ) ;
#13888=CIRCLE ( 'NONE', #3644, 6.000000000000005329 ) ;
#13921=EDGE_CURVE ( 'NONE', #9443, #15984, #24720, .T. ) ;
#13952=EDGE_CURVE ( 'NONE', #854, #24980, #15553, .T. ) ;
#13974=FACE_OUTER_BOUND ( 'NONE', #20644, .T. ) ;
#14023=AXIS2_PLACEMENT_3D ( 'NONE', #17576, #25464, #3488 ) ;
#14077=DIRECTION ( 'NONE',  ( 0.000000000000000000, -1.000000000000000000, 1.682156097916904081E-16 ) ) ;
#14246=LINE ( 'NONE', #7494, #15272 ) ;
#14248=CARTESIAN_POINT ( 'NONE',  ( 150.0000000000000284, -3.909639452396722983E-15, -7.395570986446985676E-31 ) ) ;
#14258=VERTEX_POINT ( 'NONE', #5374 ) ;
#14277=CARTESIAN_POINT ( 'NONE',  ( 190.0000000000000000, -35.78896085774750446, 65.91016826501511616 ) ) ;
#14296=VECTOR ( 'NONE', #4631, 1000.000000000000000 ) ;
#14298=CARTESIAN_POINT ( 'NONE',  ( 190.0000000000000000, -61.50000000000001421, 66.50000000000005684 ) ) ;
#14317=AXIS2_PLACEMENT_3D ( 'NONE', #2925, #23523, #13529 ) ;
#14377=CARTESIAN_POINT ( 'NONE',  ( 150.0000000000000284, -125.7889608577475116, 82.50000000000001421 ) ) ;
#14455=EDGE_LOOP ( 'NONE', ( #19267, #6106, #24770, #11923, #1661, #13687 ) ) ;
#14522=ADVANCED_FACE ( 'NONE', ( #20406 ), #16267, .F. ) ;
#14565=DIRECTION ( 'NONE',  ( 1.000000000000000000, 1.836970198721030427E-16, -0.000000000000000000 ) ) ;
#14572=SHAPE_REPRESENTATION ( 'Baseplate', ( #21058 ), #4064 ) ;
#14638=CARTESIAN_POINT ( 'NONE',  ( 190.0000000000000000, -35.78896085774750446, 82.49999999999998579 ) ) ;
#14654=CARTESIAN_POINT ( 'NONE',  ( 150.0000000000000284, -135.7889608577475258, 82.50000000000001421 ) ) ;
#14664=LINE ( 'NONE', #6553, #14920 ) ;
#14681=ADVANCED_FACE ( 'NONE', ( #7748 ), #20412, .F. ) ;
#14746=ORIENTED_EDGE ( 'NONE', *, *, #16385, .T. ) ;
#14761=ADVANCED_FACE ( 'NONE', ( #13974, #11985, #20108 ), #18226, .T. ) ;
#14899=CARTESIAN_POINT ( 'NONE',  ( 180.0000000000000000, -71.50000000000002842, -66.50000000000005684 ) ) ;
#14920=VECTOR ( 'NONE', #15065, 1000.000000000000000 ) ;
#14924=AXIS2_PLACEMENT_3D ( 'NONE', #9450, #19684, #21563 ) ;
#14973=CIRCLE ( 'NONE', #21762, 5.000000000000004441 ) ;
#14999=EDGE_CURVE ( 'NONE', #21146, #15984, #21952, .T. ) ;
#15003=EDGE_CURVE ( 'NONE', #4168, #8967, #4549, .T. ) ;
#15010=EDGE_CURVE ( 'NONE', #21905, #9342, #12377, .T. ) ;
#15043=ORIENTED_EDGE ( 'NONE', *, *, #22501, .F. ) ;
#15044=ORIENTED_EDGE ( 'NONE', *, *, #19387, .T. ) ;
#15065=DIRECTION ( 'NONE',  ( -1.303213150798907793E-16, 1.000000000000000000, -1.682156097916904081E-16 ) ) ;
#15153=VECTOR ( 'NONE', #8385, 1000.000000000000000 ) ;
#15180=ORIENTED_EDGE ( 'NONE', *, *, #5749, .F. ) ;
#15189=DIRECTION ( 'NONE',  ( 0.000000000000000000, 1.000000000000000000, 0.000000000000000000 ) ) ;
#15216=UNCERTAINTY_MEASURE_WITH_UNIT (LENGTH_MEASURE( 1.000000000000000082E-05 ), #10800, 'distance_accuracy_value', 'NONE');
#15224=DIRECTION ( 'NONE',  ( 0.000000000000000000, -1.682156097916904081E-16, -1.000000000000000000 ) ) ;
#15272=VECTOR ( 'NONE', #24509, 1000.000000000000000 ) ;
#15286=CIRCLE ( 'NONE', #1641, 5.000000000000004441 ) ;
#15297=ORIENTED_EDGE ( 'NONE', *, *, #1499, .F. ) ;
#15299=CARTESIAN_POINT ( 'NONE',  ( 180.0000000000000000, -35.78896085774750446, 65.91016826501511616 ) ) ;
#15307=CARTESIAN_POINT ( 'NONE',  ( 180.0000000000000000, -66.50000000000001421, 66.50000000000005684 ) ) ;
#15336=AXIS2_PLACEMENT_3D ( 'NONE', #23446, #1616, #9335 ) ;
#15386=CARTESIAN_POINT ( 'NONE',  ( 190.0000000000000000, -61.50000000000001421, -66.50000000000005684 ) ) ;
#15447=EDGE_CURVE ( 'NONE', #12932, #3239, #16002, .T. ) ;
#15483=ORIENTED_EDGE ( 'NONE', *, *, #3391, .F. ) ;
#15506=AXIS2_PLACEMENT_3D ( 'NONE', #878, #5505, #5379 ) ;
#15553=CIRCLE ( 'NONE', #17679, 5.000000000000004441 ) ;
#15599=FACE_BOUND ( 'NONE', #7600, .T. ) ;
#15638=DIRECTION ( 'NONE',  ( 0.000000000000000000, 0.000000000000000000, -1.000000000000000000 ) ) ;
#15677=ORIENTED_EDGE ( 'NONE', *, *, #5971, .F. ) ;
#15679=CARTESIAN_POINT ( 'NONE',  ( 190.0000000000000000, -66.50000000000001421, -66.50000000000005684 ) ) ;
#15717=STYLED_ITEM('',(#26374),#26128);
#15786=EDGE_CURVE ( 'NONE', #23734, #25845, #13888, .T. ) ;
#15809=CARTESIAN_POINT ( 'NONE',  ( 180.0000000000000000, -35.78896085774750446, 82.49999999999998579 ) ) ;
#15815=FACE_OUTER_BOUND ( 'NONE', #9093, .T. ) ;
#15852=CARTESIAN_POINT ( 'NONE',  ( 180.0000000000000000, -66.50000000000001421, 66.50000000000005684 ) ) ;
#15859=CARTESIAN_POINT ( 'NONE',  ( 160.9163046357249129, -205.7889608577475542, 55.61140153332249980 ) ) ;
#15879=PRODUCT ( 'Baseplate', 'Baseplate', '', ( #5699 ) ) ;
#15950=CYLINDRICAL_SURFACE ( 'NONE', #14924, 6.000000000000019540 ) ;
#15974=CARTESIAN_POINT ( 'NONE',  ( 180.0000000000000000, -61.50000000000001421, -66.50000000000005684 ) ) ;
#15977=DIRECTION ( 'NONE',  ( 1.000000000000000000, 0.000000000000000000, 0.000000000000000000 ) ) ;
#15984=VERTEX_POINT ( 'NONE', #3661 ) ;
#16002=CIRCLE ( 'NONE', #14317, 10.00000000000000888 ) ;
#16068=ORIENTED_EDGE ( 'NONE', *, *, #18683, .F. ) ;
#16111=DIRECTION ( 'NONE',  ( -1.000000000000000000, 0.000000000000000000, -0.000000000000000000 ) ) ;
#16204=CARTESIAN_POINT ( 'NONE',  ( 160.9163046357249129, -135.7889608577475542, 61.61140153332250691 ) ) ;
#16210=EDGE_LOOP ( 'NONE', ( #14746, #10673, #890, #15677 ) ) ;
#16267=CYLINDRICAL_SURFACE ( 'NONE', #22823, 5.000000000000004441 ) ;
#16278=ADVANCED_BREP_SHAPE_REPRESENTATION ( '', ( #26128, #21058 ), #4064 ) ;
#16337=VERTEX_POINT ( 'NONE', #14298 ) ;
#16341=EDGE_LOOP ( 'NONE', ( #15297, #25175, #17573, #24096 ) ) ;
#16385=EDGE_CURVE ( 'NONE', #2425, #3239, #10573, .T. ) ;
#16389=APPLICATION_CONTEXT ( 'automotive_design' ) ;
#16393=EDGE_CURVE ( 'NONE', #3239, #1984, #12970, .T. ) ;
#16395=VECTOR ( 'NONE', #9546, 1000.000000000000000 ) ;
#16454=ORIENTED_EDGE ( 'NONE', *, *, #21219, .F. ) ;
#16507=DIRECTION ( 'NONE',  ( 1.000000000000000000, 1.303213150798907793E-16, 2.465190328815661892E-32 ) ) ;
#16529=AXIS2_PLACEMENT_3D ( 'NONE', #18967, #8716, #25484 ) ;
#16534=FACE_OUTER_BOUND ( 'NONE', #10969, .T. ) ;
#16543=CARTESIAN_POINT ( 'NONE',  ( 190.0000000000000000, -35.78896085774750446, -65.91016826501511616 ) ) ;
#16606=AXIS2_PLACEMENT_3D ( 'NONE', #26276, #38, #8014 ) ;
#16622=AXIS2_PLACEMENT_3D ( 'NONE', #23508, #19506, #1290 ) ;
#16623=ADVANCED_FACE ( 'NONE', ( #5684, #19787, #24927 ), #575, .F. ) ;
#16661=DIRECTION ( 'NONE',  ( 0.000000000000000000, -1.000000000000000000, 0.000000000000000000 ) ) ;
#16665=CIRCLE ( 'NONE', #24748, 6.000000000000019540 ) ;
#16678=DIRECTION ( 'NONE',  ( 1.000000000000000000, 1.836970198721030427E-16, -0.000000000000000000 ) ) ;
#16697=EDGE_CURVE ( 'NONE', #25993, #6082, #19056, .T. ) ;
#16713=DIRECTION ( 'NONE',  ( 0.000000000000000000, 0.000000000000000000, 1.000000000000000000 ) ) ;
#16754=CARTESIAN_POINT ( 'NONE',  ( 180.0000000000000000, 2.292407966645821729E-14, -82.49999999999998579 ) ) ;
#16804=AXIS2_PLACEMENT_3D ( 'NONE', #15859, #22009, #5767 ) ;
#16816=ORIENTED_EDGE ( 'NONE', *, *, #24953, .F. ) ;
#16827=VECTOR ( 'NONE', #21091, 1000.000000000000000 ) ;
#16902=LINE ( 'NONE', #2542, #22951 ) ;
#17041=EDGE_LOOP ( 'NONE', ( #1901, #18273 ) ) ;
#17206=ORIENTED_EDGE ( 'NONE', *, *, #2985, .T. ) ;
#17279=DIRECTION ( 'NONE',  ( -1.303213150798907793E-16, 1.000000000000000000, -1.682156097916904081E-16 ) ) ;
#17360=ORIENTED_EDGE ( 'NONE', *, *, #15447, .F. ) ;
#17573=ORIENTED_EDGE ( 'NONE', *, *, #18926, .T. ) ;
#17575=DIRECTION ( 'NONE',  ( 0.000000000000000000, -1.000000000000000000, 0.000000000000000000 ) ) ;
#17576=CARTESIAN_POINT ( 'NONE',  ( 180.0000000000000000, -66.50000000000001421, 66.50000000000005684 ) ) ;
#17641=AXIS2_PLACEMENT_3D ( 'NONE', #1644, #10283, #18392 ) ;
#17679=AXIS2_PLACEMENT_3D ( 'NONE', #8875, #4495, #6873 ) ;
#17877=LINE ( 'NONE', #22430, #1981 ) ;
#17983=DIRECTION ( 'NONE',  ( 5.098616525425841937E-32, -2.775557561562890858E-16, -1.000000000000000000 ) ) ;
#18024=DIRECTION ( 'NONE',  ( 0.000000000000000000, 1.000000000000000000, 0.000000000000000000 ) ) ;
#18102=ORIENTED_EDGE ( 'NONE', *, *, #6961, .F. ) ;
#18134=DIRECTION ( 'NONE',  ( 0.000000000000000000, 0.000000000000000000, 1.000000000000000000 ) ) ;
#18203=CIRCLE ( 'NONE', #19484, 10.00000000000000888 ) ;
#18226=PLANE ( 'NONE',  #21533 ) ;
#18273=ORIENTED_EDGE ( 'NONE', *, *, #18926, .F. ) ;
#18345=ORIENTED_EDGE ( 'NONE', *, *, #13952, .T. ) ;
#18392=DIRECTION ( 'NONE',  ( 0.000000000000000000, -1.000000000000000000, 0.000000000000000000 ) ) ;
#18474=ORIENTED_EDGE ( 'NONE', *, *, #389, .T. ) ;
#18506=( NAMED_UNIT ( * ) SI_UNIT ( $, .STERADIAN. ) SOLID_ANGLE_UNIT ( ) );
#18507=EDGE_LOOP ( 'NONE', ( #8759, #4134, #6537, #11333, #18979, #21680, #15180, #13306 ) ) ;
#18529=DIRECTION ( 'NONE',  ( 0.000000000000000000, 1.000000000000000000, 0.000000000000000000 ) ) ;
#18535=CARTESIAN_POINT ( 'NONE',  ( 190.0000000000000000, -35.78896085774753288, 1.496915739050593134E-14 ) ) ;
#18586=EDGE_CURVE ( 'NONE', #22454, #12932, #20952, .T. ) ;
#18648=ORIENTED_EDGE ( 'NONE', *, *, #5971, .T. ) ;
#18651=LINE ( 'NONE', #8808, #26003 ) ;
#18683=EDGE_CURVE ( 'NONE', #3723, #20976, #16665, .T. ) ;
#18741=DIRECTION ( 'NONE',  ( 0.000000000000000000, -1.000000000000000000, 0.000000000000000000 ) ) ;
#18794=DIRECTION ( 'NONE',  ( 1.303213150798907793E-16, -1.000000000000000000, 2.775557561562890858E-16 ) ) ;
#18848=ORIENTED_EDGE ( 'NONE', *, *, #2985, .F. ) ;
#18915=ORIENTED_EDGE ( 'NONE', *, *, #5749, .T. ) ;
#18926=EDGE_CURVE ( 'NONE', #14258, #22079, #1799, .T. ) ;
#18967=CARTESIAN_POINT ( 'NONE',  ( 180.0000000000000000, -66.50000000000001421, -66.50000000000005684 ) ) ;
#18979=ORIENTED_EDGE ( 'NONE', *, *, #11905, .T. ) ;
#19009=ORIENTED_EDGE ( 'NONE', *, *, #3876, .F. ) ;
#19052=CARTESIAN_POINT ( 'NONE',  ( 180.0000000000000000, -35.78896085774750446, 65.91016826501511616 ) ) ;
#19056=LINE ( 'NONE', #4571, #20228 ) ;
#19135=CARTESIAN_POINT ( 'NONE',  ( 160.9163046357249129, -205.7889608577475542, 55.61140153332249980 ) ) ;
#19170=( LENGTH_UNIT ( ) NAMED_UNIT ( * ) SI_UNIT ( .MILLI., .METRE. ) );
#19201=CARTESIAN_POINT ( 'NONE',  ( 180.0000000000000000, -71.50000000000002842, 66.50000000000005684 ) ) ;
#19267=ORIENTED_EDGE ( 'NONE', *, *, #16697, .T. ) ;
#19293=CARTESIAN_POINT ( 'NONE',  ( 160.9163046357249129, -205.7889608577475542, 49.61140153332248559 ) ) ;
#19313=CARTESIAN_POINT ( 'NONE',  ( 190.0000000000000000, -35.78896085774750446, -82.49999999999998579 ) ) ;
#19387=EDGE_CURVE ( 'NONE', #24980, #23006, #9218, .T. ) ;
#19395=EDGE_CURVE ( 'NONE', #10429, #9342, #9091, .T. ) ;
#19420=( NAMED_UNIT ( * ) SI_UNIT ( $, .STERADIAN. ) SOLID_ANGLE_UNIT ( ) );
#19451=CARTESIAN_POINT ( 'NONE',  ( 180.0000000000000000, -71.50000000000002842, -66.50000000000005684 ) ) ;
#19484=AXIS2_PLACEMENT_3D ( 'NONE', #6283, #2174, #22663 ) ;
#19486=EDGE_CURVE ( 'NONE', #22320, #10668, #14973, .T. ) ;
#19506=DIRECTION ( 'NONE',  ( -1.836970198721030427E-16, 1.000000000000000000, -1.682156097916904081E-16 ) ) ;
#19510=ORIENTED_EDGE ( 'NONE', *, *, #14999, .T. ) ;
#19555=DIRECTION ( 'NONE',  ( 0.000000000000000000, -1.000000000000000000, 0.000000000000000000 ) ) ;
#19579=CARTESIAN_POINT ( 'NONE',  ( 180.0000000000000284, -115.7889608577475400, 1.947751065783218452E-14 ) ) ;
#19587=ORIENTED_EDGE ( 'NONE', *, *, #23125, .T. ) ;
#19624=DIRECTION ( 'NONE',  ( -1.000000000000000000, 0.000000000000000000, 0.000000000000000000 ) ) ;
#19629=EDGE_CURVE ( 'NONE', #854, #20872, #5875, .T. ) ;
#19638=FACE_BOUND ( 'NONE', #21082, .T. ) ;
#19684=DIRECTION ( 'NONE',  ( -1.303213150798907793E-16, 1.000000000000000000, -1.682156097916904081E-16 ) ) ;
#19787=FACE_BOUND ( 'NONE', #5079, .T. ) ;
#19888=DIRECTION ( 'NONE',  ( -1.836970198721030427E-16, 1.000000000000000000, -1.682156097916904327E-16 ) ) ;
#19946=LINE ( 'NONE', #1730, #7697 ) ;
#19976=CARTESIAN_POINT ( 'NONE',  ( 160.9163046357249129, -135.7889608577475542, 49.61140153332247138 ) ) ;
#20086=LINE ( 'NONE', #6111, #10459 ) ;
#20108=FACE_BOUND ( 'NONE', #21334, .T. ) ;
#20220=VECTOR ( 'NONE', #983, 1000.000000000000000 ) ;
#20228=VECTOR ( 'NONE', #18794, 1000.000000000000000 ) ;
#20369=CARTESIAN_POINT ( 'NONE',  ( 150.0000000000000284, -125.7889608577475400, -82.49999999999998579 ) ) ;
#20406=FACE_OUTER_BOUND ( 'NONE', #693, .T. ) ;
#20412=CYLINDRICAL_SURFACE ( 'NONE', #24536, 6.000000000000019540 ) ;
#20425=CARTESIAN_POINT ( 'NONE',  ( 180.0000000000000000, -35.78896085774750446, -82.49999999999998579 ) ) ;
#20505=DIRECTION ( 'NONE',  ( 1.303213150798907793E-16, -1.000000000000000000, 2.775557561562890858E-16 ) ) ;
#20531=CARTESIAN_POINT ( 'NONE',  ( 190.0000000000000284, -125.7889608577475684, -82.49999999999998579 ) ) ;
#20634=DIRECTION ( 'NONE',  ( -1.000000000000000000, -1.303213150798907793E-16, -2.465190328815661892E-32 ) ) ;
#20644=EDGE_LOOP ( 'NONE', ( #18915, #8602, #22481, #7955, #19510, #13310 ) ) ;
#20666=AXIS2_PLACEMENT_3D ( 'NONE', #2032, #3614, #6142 ) ;
#20743=ORIENTED_EDGE ( 'NONE', *, *, #795, .T. ) ;
#20749=EDGE_LOOP ( 'NONE', ( #24955, #9097, #16454, #9471 ) ) ;
#20832=FACE_OUTER_BOUND ( 'NONE', #10860, .T. ) ;
#20872=VERTEX_POINT ( 'NONE', #15386 ) ;
#20880=ADVANCED_FACE ( 'NONE', ( #19638, #3162, #25520 ), #3286, .F. ) ;
#20895=PLANE ( 'NONE',  #8731 ) ;
#20916=ORIENTED_EDGE ( 'NONE', *, *, #19629, .T. ) ;
#20952=LINE ( 'NONE', #12689, #6460 ) ;
#20976=VERTEX_POINT ( 'NONE', #8143 ) ;
#21058=AXIS2_PLACEMENT_3D ( 'NONE', #7994, #22, #15977 ) ;
#21082=EDGE_LOOP ( 'NONE', ( #6530, #9874 ) ) ;
#21088=VECTOR ( 'NONE', #17279, 1000.000000000000000 ) ;
#21091=DIRECTION ( 'NONE',  ( -4.657398277317547006E-32, 1.682156097916904081E-16, 1.000000000000000000 ) ) ;
#21130=CARTESIAN_POINT ( 'NONE',  ( 160.9163046357249129, -135.7889608577475542, -55.61140153332245006 ) ) ;
#21143=FACE_OUTER_BOUND ( 'NONE', #6240, .T. ) ;
#21146=VERTEX_POINT ( 'NONE', #19052 ) ;
#21169=ORIENTED_EDGE ( 'NONE', *, *, #10101, .F. ) ;
#21190=CARTESIAN_POINT ( 'NONE',  ( 190.0000000000000000, -66.50000000000001421, 66.50000000000005684 ) ) ;
#21194=DIRECTION ( 'NONE',  ( 1.000000000000000000, 1.836970198721030427E-16, -0.000000000000000000 ) ) ;
#21219=EDGE_CURVE ( 'NONE', #21905, #21146, #18651, .T. ) ;
#21327=LINE ( 'NONE', #13083, #393 ) ;
#21334=EDGE_LOOP ( 'NONE', ( #18345, #20743 ) ) ;
#21349=EDGE_CURVE ( 'NONE', #20872, #23006, #12390, .T. ) ;
#21360=FACE_OUTER_BOUND ( 'NONE', #1245, .T. ) ;
#21371=VERTEX_POINT ( 'NONE', #21431 ) ;
#21431=CARTESIAN_POINT ( 'NONE',  ( 169.9999999999999716, -125.7889608577475400, -82.49999999999998579 ) ) ;
#21465=MECHANICAL_DESIGN_GEOMETRIC_PRESENTATION_REPRESENTATION('',(#15717),#222);
#21533=AXIS2_PLACEMENT_3D ( 'NONE', #2815, #20634, #12646 ) ;
#21563=DIRECTION ( 'NONE',  ( 0.000000000000000000, 0.000000000000000000, 1.000000000000000000 ) ) ;
#21572=PLANE ( 'NONE',  #15336 ) ;
#21668=CYLINDRICAL_SURFACE ( 'NONE', #12294, 10.00000000000000888 ) ;
#21680=ORIENTED_EDGE ( 'NONE', *, *, #9879, .T. ) ;
#21716=CIRCLE ( 'NONE', #8108, 6.000000000000019540 ) ;
#21735=FACE_OUTER_BOUND ( 'NONE', #2757, .T. ) ;
#21762=AXIS2_PLACEMENT_3D ( 'NONE', #3231, #9468, #17575 ) ;
#21816=EDGE_CURVE ( 'NONE', #4168, #5362, #19946, .T. ) ;
#21859=DIRECTION ( 'NONE',  ( 0.000000000000000000, 1.000000000000000000, 0.000000000000000000 ) ) ;
#21905=VERTEX_POINT ( 'NONE', #15809 ) ;
#21952=CIRCLE ( 'NONE', #3268, 74.99999999999995737 ) ;
#21996=DIRECTION ( 'NONE',  ( 0.000000000000000000, -1.000000000000000000, 0.000000000000000000 ) ) ;
#22009=DIRECTION ( 'NONE',  ( -1.303213150798907793E-16, 1.000000000000000000, -1.682156097916904081E-16 ) ) ;
#22072=PRODUCT_DEFINITION_SHAPE ( 'NONE', 'NONE',  #11592 ) ;
#22074=ORIENTED_EDGE ( 'NONE', *, *, #24254, .T. ) ;
#22079=VERTEX_POINT ( 'NONE', #23146 ) ;
#22097=AXIS2_PLACEMENT_3D ( 'NONE', #11348, #5624, #21996 ) ;
#22116=CARTESIAN_POINT ( 'NONE',  ( 190.0000000000000000, -71.50000000000002842, 66.50000000000005684 ) ) ;
#22208=CARTESIAN_POINT ( 'NONE',  ( 180.0000000000000000, -35.78896085774753288, 1.496915739050593134E-14 ) ) ;
#22320=VERTEX_POINT ( 'NONE', #25700 ) ;
#22333=AXIS2_PLACEMENT_3D ( 'NONE', #3511, #9626, #15224 ) ;
#22404=CARTESIAN_POINT ( 'NONE',  ( 169.9999999999999716, -115.7889608577475258, 82.50000000000000000 ) ) ;
#22411=VECTOR ( 'NONE', #20505, 1000.000000000000000 ) ;
#22430=CARTESIAN_POINT ( 'NONE',  ( 180.0000000000000000, 2.292407966645821729E-14, -82.49999999999998579 ) ) ;
#22454=VERTEX_POINT ( 'NONE', #19313 ) ;
#22481=ORIENTED_EDGE ( 'NONE', *, *, #15010, .F. ) ;
#22501=EDGE_CURVE ( 'NONE', #8967, #21371, #3564, .T. ) ;
#22525=ORIENTED_EDGE ( 'NONE', *, *, #795, .F. ) ;
#22535=CYLINDRICAL_SURFACE ( 'NONE', #2627, 5.000000000000004441 ) ;
#22542=LINE ( 'NONE', #18535, #1086 ) ;
#22619=VECTOR ( 'NONE', #11455, 1000.000000000000000 ) ;
#22663=DIRECTION ( 'NONE',  ( 1.000000000000000000, 0.000000000000000000, 0.000000000000000000 ) ) ;
#22777=SHAPE_REPRESENTATION_RELATIONSHIP ( 'NONE' , 'NONE' ,  #14572, #16278 ) ;
#22798=CARTESIAN_POINT ( 'NONE',  ( 180.0000000000000000, -61.50000000000001421, -66.50000000000005684 ) ) ;
#22818=ORIENTED_EDGE ( 'NONE', *, *, #21816, .T. ) ;
#22823=AXIS2_PLACEMENT_3D ( 'NONE', #15852, #10018, #21859 ) ;
#22951=VECTOR ( 'NONE', #12507, 1000.000000000000000 ) ;
#23006=VERTEX_POINT ( 'NONE', #11069 ) ;
#23028=DIRECTION ( 'NONE',  ( 0.000000000000000000, 0.000000000000000000, 1.000000000000000000 ) ) ;
#23100=CYLINDRICAL_SURFACE ( 'NONE', #16529, 5.000000000000004441 ) ;
#23125=EDGE_CURVE ( 'NONE', #10668, #22320, #3849, .T. ) ;
#23146=CARTESIAN_POINT ( 'NONE',  ( 160.9163046357249129, -125.7889608577475684, -49.61140153332242875 ) ) ;
#23153=FACE_OUTER_BOUND ( 'NONE', #18507, .T. ) ;
#23167=ORIENTED_EDGE ( 'NONE', *, *, #18683, .T. ) ;
#23266=ORIENTED_EDGE ( 'NONE', *, *, #13921, .T. ) ;
#23309=DIRECTION ( 'NONE',  ( 0.000000000000000000, -1.000000000000000000, 0.000000000000000000 ) ) ;
#23317=DIRECTION ( 'NONE',  ( 1.000000000000000000, 1.303213150798907793E-16, 2.465190328815661892E-32 ) ) ;
#23437=CARTESIAN_POINT ( 'NONE',  ( 180.0000000000000000, -35.78896085774750446, 82.49999999999998579 ) ) ;
#23446=CARTESIAN_POINT ( 'NONE',  ( 180.0000000000000000, 4.582242954935206147E-14, 82.49999999999997158 ) ) ;
#23465=ORIENTED_EDGE ( 'NONE', *, *, #6633, .T. ) ;
#23508=CARTESIAN_POINT ( 'NONE',  ( 180.0000000000000284, -135.7889608577475542, 2.284182285366599633E-14 ) ) ;
#23523=DIRECTION ( 'NONE',  ( -0.000000000000000000, -0.000000000000000000, -1.000000000000000000 ) ) ;
#23580=ORIENTED_EDGE ( 'NONE', *, *, #14999, .F. ) ;
#23621=ADVANCED_FACE ( 'NONE', ( #1451 ), #25801, .F. ) ;
#23636=VERTEX_POINT ( 'NONE', #9686 ) ;
#23687=ADVANCED_FACE ( 'NONE', ( #26342 ), #21668, .T. ) ;
#23705=ORIENTED_EDGE ( 'NONE', *, *, #10042, .T. ) ;
#23724=FACE_BOUND ( 'NONE', #17041, .T. ) ;
#23734=VERTEX_POINT ( 'NONE', #16204 ) ;
#23782=CARTESIAN_POINT ( 'NONE',  ( 180.0000000000000000, -35.78896085774750446, -82.49999999999998579 ) ) ;
#23792=AXIS2_PLACEMENT_3D ( 'NONE', #14248, #16111, #7854 ) ;
#23804=DIRECTION ( 'NONE',  ( 1.000000000000000000, 1.303213150798907793E-16, 2.465190328815661892E-32 ) ) ;
#23836=AXIS2_PLACEMENT_3D ( 'NONE', #24089, #6386, #5864 ) ;
#23907=CARTESIAN_POINT ( 'NONE',  ( 180.0000000000000000, -61.50000000000001421, 66.50000000000005684 ) ) ;
#24044=CLOSED_SHELL ( 'NONE', ( #7117, #14681, #13218, #14522, #12243, #23621, #13220, #12560, #2598, #25407, #20880, #11346, #14761, #16623, #1764, #25604, #23687, #3149, #4604, #1819 ) ) ;
#24052=DIRECTION ( 'NONE',  ( 4.657398277317546459E-32, -1.682156097916904081E-16, -1.000000000000000000 ) ) ;
#24089=CARTESIAN_POINT ( 'NONE',  ( 180.0000000000000000, -35.78896085774753288, -1.496915739050591872E-14 ) ) ;
#24096=ORIENTED_EDGE ( 'NONE', *, *, #11906, .F. ) ;
#24132=CARTESIAN_POINT ( 'NONE',  ( 160.9163046357249129, -205.7889608577475542, -55.61140153332243585 ) ) ;
#24193=CARTESIAN_POINT ( 'NONE',  ( 180.0000000000000284, -125.7889608577475400, 2.115966675574909200E-14 ) ) ;
#24254=EDGE_CURVE ( 'NONE', #5362, #2425, #14246, .T. ) ;
#24342=ORIENTED_EDGE ( 'NONE', *, *, #21349, .F. ) ;
#24383=ORIENTED_EDGE ( 'NONE', *, *, #6633, .F. ) ;
#24504=CARTESIAN_POINT ( 'NONE',  ( 180.0000000000000000, 6.980486755139914804E-14, 0.000000000000000000 ) ) ;
#24509=DIRECTION ( 'NONE',  ( -0.000000000000000000, -1.000000000000000000, -0.000000000000000000 ) ) ;
#24525=CARTESIAN_POINT ( 'NONE',  ( 169.9999999999999716, -125.7889608577475116, 82.50000000000001421 ) ) ;
#24536=AXIS2_PLACEMENT_3D ( 'NONE', #24132, #12021, #18134 ) ;
#24556=DIRECTION ( 'NONE',  ( 1.000000000000000000, 1.836970198721030427E-16, -0.000000000000000000 ) ) ;
#24577=EDGE_LOOP ( 'NONE', ( #22525, #15044, #11556, #6832 ) ) ;
#24662=FACE_OUTER_BOUND ( 'NONE', #24577, .T. ) ;
#24680=ORIENTED_EDGE ( 'NONE', *, *, #4973, .F. ) ;
#24720=LINE ( 'NONE', #6476, #14296 ) ;
#24748=AXIS2_PLACEMENT_3D ( 'NONE', #4725, #25080, #6831 ) ;
#24770=ORIENTED_EDGE ( 'NONE', *, *, #18586, .F. ) ;
#24793=LINE ( 'NONE', #14654, #11888 ) ;
#24796=CARTESIAN_POINT ( 'NONE',  ( 180.0000000000000000, -66.50000000000001421, -66.50000000000005684 ) ) ;
#24927=FACE_BOUND ( 'NONE', #12350, .T. ) ;
#24953=EDGE_CURVE ( 'NONE', #6082, #12932, #16902, .T. ) ;
#24955=ORIENTED_EDGE ( 'NONE', *, *, #2313, .T. ) ;
#24980=VERTEX_POINT ( 'NONE', #14899 ) ;
#25080=DIRECTION ( 'NONE',  ( -1.303213150798907793E-16, 1.000000000000000000, -1.682156097916904081E-16 ) ) ;
#25081=ORIENTED_EDGE ( 'NONE', *, *, #2098, .T. ) ;
#25175=ORIENTED_EDGE ( 'NONE', *, *, #12062, .T. ) ;
#25251=CIRCLE ( 'NONE', #11622, 5.000000000000004441 ) ;
#25351=EDGE_CURVE ( 'NONE', #15984, #4199, #459, .T. ) ;
#25385=DIRECTION ( 'NONE',  ( -1.000000000000000000, 0.000000000000000000, 0.000000000000000000 ) ) ;
#25407=ADVANCED_FACE ( 'NONE', ( #1627 ), #1371, .F. ) ;
#25425=EDGE_LOOP ( 'NONE', ( #19587, #8940 ) ) ;
#25464=DIRECTION ( 'NONE',  ( 1.000000000000000000, 1.836970198721030427E-16, -0.000000000000000000 ) ) ;
#25476=PRODUCT_DEFINITION_CONTEXT ( 'detailed design', #11214, 'design' ) ;
#25484=DIRECTION ( 'NONE',  ( 0.000000000000000000, 1.000000000000000000, 0.000000000000000000 ) ) ;
#25503=VECTOR ( 'NONE', #11194, 1000.000000000000000 ) ;
#25520=FACE_OUTER_BOUND ( 'NONE', #16210, .T. ) ;
#25524=ORIENTED_EDGE ( 'NONE', *, *, #10438, .F. ) ;
#25551=ORIENTED_EDGE ( 'NONE', *, *, #13952, .F. ) ;
#25591=DIRECTION ( 'NONE',  ( -4.657398277317546459E-32, 1.682156097916904081E-16, 1.000000000000000000 ) ) ;
#25604=ADVANCED_FACE ( 'NONE', ( #26115 ), #9866, .T. ) ;
#25700=CARTESIAN_POINT ( 'NONE',  ( 180.0000000000000000, -71.50000000000002842, 66.50000000000005684 ) ) ;
#25703=FACE_OUTER_BOUND ( 'NONE', #3957, .T. ) ;
#25788=UNCERTAINTY_MEASURE_WITH_UNIT (LENGTH_MEASURE( 1.000000000000000082E-05 ), #19170, 'distance_accuracy_value', 'NONE');
#25801=PLANE ( 'NONE',  #13555 ) ;
#25804=VERTEX_POINT ( 'NONE', #22116 ) ;
#25845=VERTEX_POINT ( 'NONE', #19976 ) ;
#25933=CARTESIAN_POINT ( 'NONE',  ( 169.9999999999999716, -125.7889608577475116, 82.50000000000001421 ) ) ;
#25964=LINE ( 'NONE', #23437, #25503 ) ;
#25982=DIRECTION ( 'NONE',  ( 1.000000000000000000, 1.836970198721030427E-16, -0.000000000000000000 ) ) ;
#25993=VERTEX_POINT ( 'NONE', #14638 ) ;
#26003=VECTOR ( 'NONE', #6805, 1000.000000000000000 ) ;
#26029=CARTESIAN_POINT ( 'NONE',  ( 160.9163046357249129, -135.7889608577475542, 55.61140153332248559 ) ) ;
#26035=DIRECTION ( 'NONE',  ( 1.000000000000000000, 1.836970198721030427E-16, -0.000000000000000000 ) ) ;
#26070=DIRECTION ( 'NONE',  ( 1.836970198721030427E-16, -1.000000000000000000, 4.182618615277681568E-16 ) ) ;
#26115=FACE_OUTER_BOUND ( 'NONE', #4459, .T. ) ;
#26128=MANIFOLD_SOLID_BREP ( 'Cut-Extrude5', #24044 ) ;
#26219=ORIENTED_EDGE ( 'NONE', *, *, #4923, .F. ) ;
#26276=CARTESIAN_POINT ( 'NONE',  ( 160.9163046357249129, -135.7889608577475542, 55.61140153332248559 ) ) ;
#26322=ORIENTED_EDGE ( 'NONE', *, *, #7759, .T. ) ;
#26342=FACE_OUTER_BOUND ( 'NONE', #10399, .T. ) ;
#26368=COLOUR_RGB('Dark Blue',0.08,0.2,0.34);
#26369=FILL_AREA_STYLE_COLOUR('',#26368);
#26370=FILL_AREA_STYLE('',(#26369));
#26371=SURFACE_STYLE_FILL_AREA(#26370);
#26372=SURFACE_SIDE_STYLE('',(#26371));
#26373=SURFACE_STYLE_USAGE(.BOTH.,#26372);
#26374=PRESENTATION_STYLE_ASSIGNMENT((#26373));
ENDSEC;
END-ISO-10303-21;
